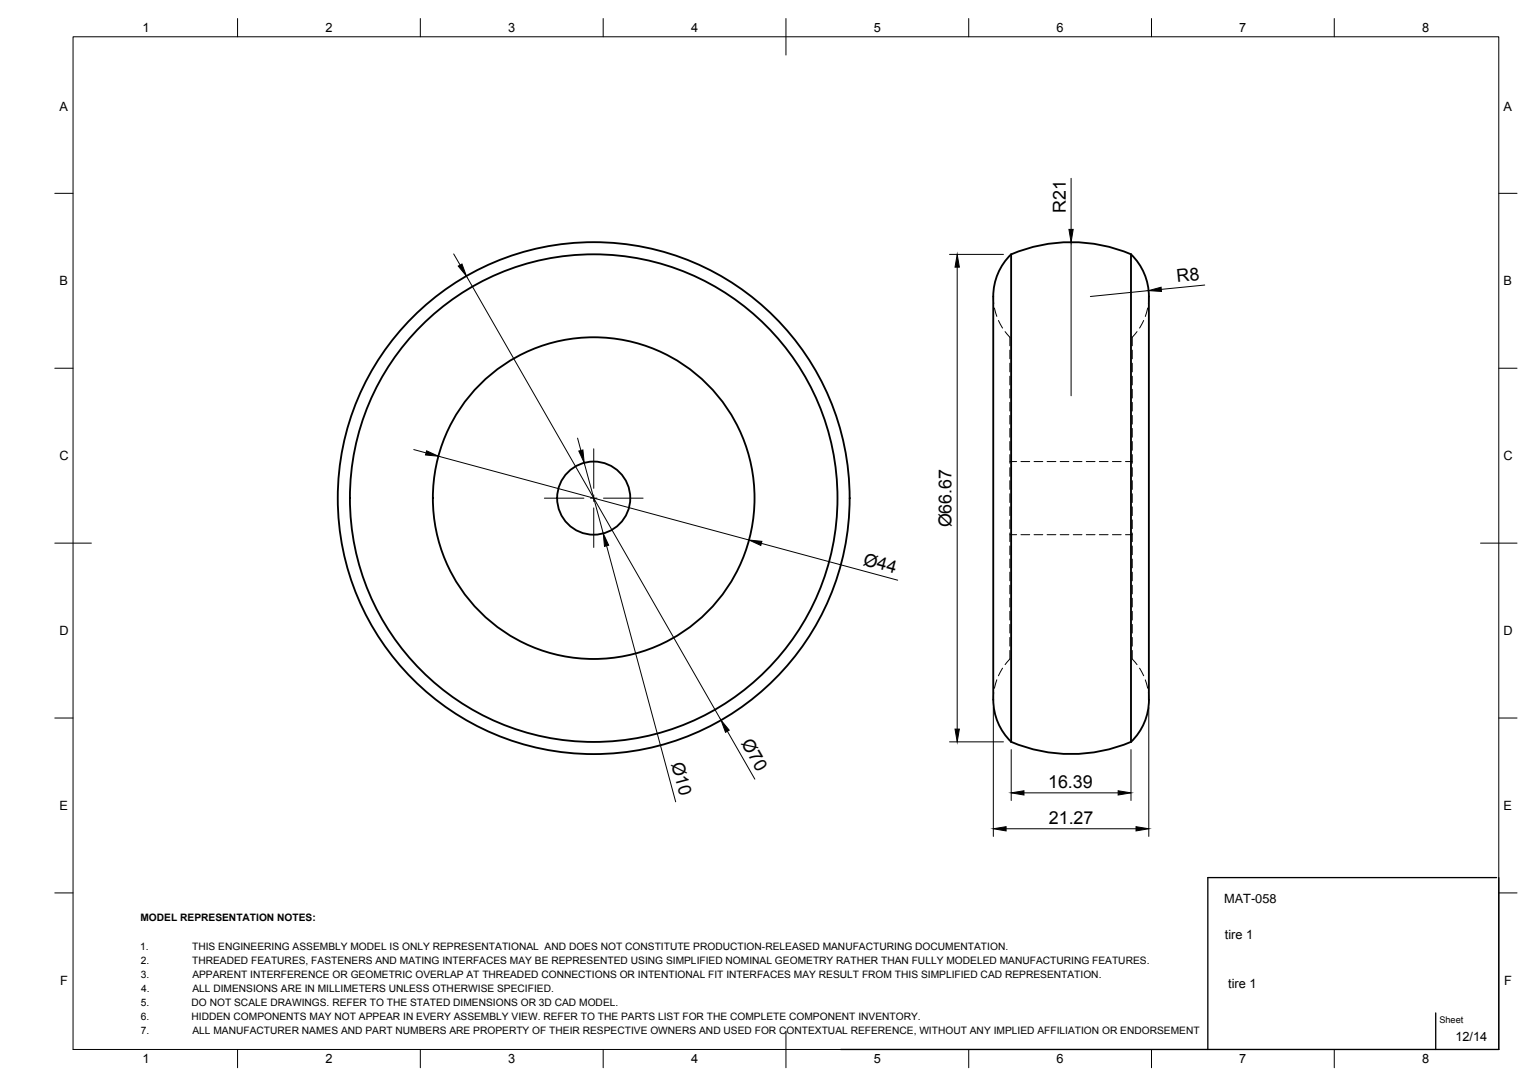
ISO-10303-21;
HEADER;
FILE_DESCRIPTION (('STEP AP214'),
    '1' );
FILE_NAME ('tire 1.step',
    '2026-10-21T17:54:40',
    ( '' ),
    ( '' ),
    'SwSTEP 2.0',
    'SolidWorks 2026',
    '' );
FILE_SCHEMA (( 'AUTOMOTIVE_DESIGN' ));
ENDSEC;

DATA;
#3=ORIENTED_EDGE ( 'NONE', *, *, #134, .T. ) ;
#134=EDGE_CURVE ( 'NONE', #24013, #25229, #8136, .T. ) ;
#450=PRODUCT_DEFINITION_FORMATION_WITH_SPECIFIED_SOURCE ( 'ANY', '', #29832, .NOT_KNOWN. ) ;
#461=DIRECTION ( 'NONE',  ( -1.000000000000000000, -0.000000000000000000, -0.000000000000000000 ) ) ;
#822=DIRECTION ( 'NONE',  ( -1.000000000000000000, -0.000000000000000000, -0.000000000000000000 ) ) ;
#883=ADVANCED_FACE ( 'NONE', ( #35791 ), #3095, .T. ) ;
#885=AXIS2_PLACEMENT_3D ( 'NONE', #24920, #14879, #22568 ) ;
#1237=VERTEX_POINT ( 'NONE', #11074 ) ;
#1353=DIRECTION ( 'NONE',  ( 0.000000000000000000, -1.224646799147352961E-16, 1.000000000000000000 ) ) ;
#1445=FACE_OUTER_BOUND ( 'NONE', #37012, .T. ) ;
#1633=CIRCLE ( 'NONE', #43400, 22.00000000000000000 ) ;
#1686=DIRECTION ( 'NONE',  ( -1.000000000000000000, -0.000000000000000000, -0.000000000000000000 ) ) ;
#2253=ORIENTED_EDGE ( 'NONE', *, *, #43738, .T. ) ;
#3057=DIRECTION ( 'NONE',  ( 0.000000000000000000, 0.000000000000000000, 1.000000000000000000 ) ) ;
#3095=TOROIDAL_SURFACE ( 'NONE', #31808, 27.58190990837850265, 8.000000000000000000 ) ;
#3153=CLOSED_SHELL ( 'NONE', ( #5898, #9220, #18286, #37671, #20586, #18104, #14876, #883, #26048, #41307 ) ) ;
#3617=CARTESIAN_POINT ( 'NONE',  ( -1.642172164747307761, 0.000000000000000000, 27.58190990837850265 ) ) ;
#3941=EDGE_CURVE ( 'NONE', #40207, #1237, #47400, .T. ) ;
#4194=VERTEX_POINT ( 'NONE', #39222 ) ;
#4266=( LENGTH_UNIT ( ) NAMED_UNIT ( * ) SI_UNIT ( .MILLI., .METRE. ) );
#4521=DIRECTION ( 'NONE',  ( 0.000000000000000000, 0.000000000000000000, -1.000000000000000000 ) ) ;
#4589=AXIS2_PLACEMENT_3D ( 'NONE', #21174, #1686, #4521 ) ;
#4597=DIRECTION ( 'NONE',  ( 0.000000000000000000, 0.000000000000000000, 1.000000000000000000 ) ) ;
#4997=VERTEX_POINT ( 'NONE', #45113 ) ;
#5069=DIRECTION ( 'NONE',  ( 0.000000000000000000, 0.000000000000000000, -1.000000000000000000 ) ) ;
#5073=UNCERTAINTY_MEASURE_WITH_UNIT (LENGTH_MEASURE( 1.000000000000000082E-05 ), #4266, 'distance_accuracy_value', 'NONE');
#5186=CARTESIAN_POINT ( 'NONE',  ( 3.627208138665139803, 3.377809768366639828E-15, -27.58190990837850265 ) ) ;
#5215=DIRECTION ( 'NONE',  ( -0.000000000000000000, 0.000000000000000000, 1.000000000000000000 ) ) ;
#5308=AXIS2_PLACEMENT_3D ( 'NONE', #16570, #47819, #12711 ) ;
#5438=DIRECTION ( 'NONE',  ( 0.000000000000000000, 0.000000000000000000, -1.000000000000000000 ) ) ;
#5528=DIRECTION ( 'NONE',  ( 0.000000000000000000, -1.224646799147352961E-16, 1.000000000000000000 ) ) ;
#5532=MANIFOLD_SOLID_BREP ( 'Cut-Extrude1', #3153 ) ;
#5590=VERTEX_POINT ( 'NONE', #17317 ) ;
#5840=CARTESIAN_POINT ( 'NONE',  ( -7.372990760266265653, 0.000000000000000000, 0.000000000000000000 ) ) ;
#5898=ADVANCED_FACE ( 'NONE', ( #44142 ), #37251, .F. ) ;
#5914=ORIENTED_EDGE ( 'NONE', *, *, #13078, .F. ) ;
#6211=DIRECTION ( 'NONE',  ( 1.000000000000000000, 0.000000000000000000, 0.000000000000000000 ) ) ;
#6301=ADVANCED_BREP_SHAPE_REPRESENTATION ( '', ( #5532, #45486 ), #38984 ) ;
#6304=DIRECTION ( 'NONE',  ( -1.000000000000000000, -0.000000000000000000, -0.000000000000000000 ) ) ;
#6817=TOROIDAL_SURFACE ( 'NONE', #21572, 27.58190990837850265, 8.000000000000000000 ) ;
#7306=AXIS2_PLACEMENT_3D ( 'NONE', #34640, #28697, #4597 ) ;
#7375=CIRCLE ( 'NONE', #12277, 20.99999999999999289 ) ;
#7527=ORIENTED_EDGE ( 'NONE', *, *, #40856, .T. ) ;
#7765=TOROIDAL_SURFACE ( 'NONE', #29871, 27.58190990837850265, 8.000000000000000000 ) ;
#7813=DIRECTION ( 'NONE',  ( 0.000000000000000000, 0.000000000000000000, 1.000000000000000000 ) ) ;
#8136=CIRCLE ( 'NONE', #47408, 8.000000000000000000 ) ;
#8438=SHAPE_REPRESENTATION ( 'tire 1', ( #45486 ), #38984 ) ;
#8740=CARTESIAN_POINT ( 'NONE',  ( -9.643172164747307207, 6.123233995736766282E-16, 5.000000000000000000 ) ) ;
#9130=DIRECTION ( 'NONE',  ( -0.000000000000000000, 1.000000000000000000, 1.224646799147353207E-16 ) ) ;
#9177=DIRECTION ( 'NONE',  ( 0.000000000000000000, 0.000000000000000000, 1.000000000000000000 ) ) ;
#9220=ADVANCED_FACE ( 'NONE', ( #49094 ), #40899, .T. ) ;
#9304=DIRECTION ( 'NONE',  ( 0.000000000000000000, -1.224646799147353207E-16, 1.000000000000000000 ) ) ;
#9319=FACE_OUTER_BOUND ( 'NONE', #17798, .T. ) ;
#9347=CARTESIAN_POINT ( 'NONE',  ( 9.358026734184097251, 0.000000000000000000, 0.000000000000000000 ) ) ;
#9413=AXIS2_PLACEMENT_3D ( 'NONE', #43306, #23048, #38978 ) ;
#9443=CARTESIAN_POINT ( 'NONE',  ( -7.200076171898729172, 0.000000000000000000, 0.000000000000000000 ) ) ;
#9886=CARTESIAN_POINT ( 'NONE',  ( 3.627208138665139803, 0.000000000000000000, 0.000000000000000000 ) ) ;
#10134=DIRECTION ( 'NONE',  ( 0.000000000000000000, 0.000000000000000000, 1.000000000000000000 ) ) ;
#10168=EDGE_CURVE ( 'NONE', #20400, #29240, #39842, .T. ) ;
#10474=ORIENTED_EDGE ( 'NONE', *, *, #35944, .F. ) ;
#10579=ORIENTED_EDGE ( 'NONE', *, *, #30205, .T. ) ;
#10812=DIRECTION ( 'NONE',  ( 0.000000000000000000, -1.000000000000000000, 0.000000000000000000 ) ) ;
#10904=APPLICATION_CONTEXT ( 'automotive_design' ) ;
#11038=ORIENTED_EDGE ( 'NONE', *, *, #30205, .F. ) ;
#11074=CARTESIAN_POINT ( 'NONE',  ( 9.185112145816566098, 4.082484168683570285E-15, -33.33601305720110020 ) ) ;
#11289=ORIENTED_EDGE ( 'NONE', *, *, #10168, .F. ) ;
#11709=EDGE_CURVE ( 'NONE', #29240, #1237, #26209, .T. ) ;
#11747=DIRECTION ( 'NONE',  ( 0.000000000000000000, 0.000000000000000000, 1.000000000000000000 ) ) ;
#11876=ORIENTED_EDGE ( 'NONE', *, *, #31746, .T. ) ;
#11930=DIRECTION ( 'NONE',  ( 0.000000000000000000, 0.000000000000000000, 1.000000000000000000 ) ) ;
#12005=AXIS2_PLACEMENT_3D ( 'NONE', #25454, #6211, #5438 ) ;
#12277=AXIS2_PLACEMENT_3D ( 'NONE', #28780, #44156, #37267 ) ;
#12476=MECHANICAL_DESIGN_GEOMETRIC_PRESENTATION_REPRESENTATION('',(#29698),#31333);
#12652=PLANE ( 'NONE',  #34799 ) ;
#12682=DIRECTION ( 'NONE',  ( -1.000000000000000000, -0.000000000000000000, -0.000000000000000000 ) ) ;
#12711=DIRECTION ( 'NONE',  ( 0.000000000000000000, 0.000000000000000000, -1.000000000000000000 ) ) ;
#13023=DIRECTION ( 'NONE',  ( -1.000000000000000000, -0.000000000000000000, -0.000000000000000000 ) ) ;
#13078=EDGE_CURVE ( 'NONE', #24013, #18422, #22060, .T. ) ;
#13189=DIRECTION ( 'NONE',  ( 0.000000000000000000, 0.000000000000000000, 1.000000000000000000 ) ) ;
#13288=ORIENTED_EDGE ( 'NONE', *, *, #16440, .F. ) ;
#13319=DIRECTION ( 'NONE',  ( 0.000000000000000000, 0.000000000000000000, 1.000000000000000000 ) ) ;
#13923=EDGE_CURVE ( 'NONE', #29240, #20400, #26964, .T. ) ;
#14061=DIRECTION ( 'NONE',  ( 0.000000000000000000, 0.000000000000000000, 1.000000000000000000 ) ) ;
#14081=CARTESIAN_POINT ( 'NONE',  ( -7.200076171898729172, 0.000000000000000000, 33.33601305720110020 ) ) ;
#14551=ORIENTED_EDGE ( 'NONE', *, *, #29009, .T. ) ;
#14825=ORIENTED_EDGE ( 'NONE', *, *, #35307, .F. ) ;
#14876=ADVANCED_FACE ( 'NONE', ( #19865 ), #22959, .T. ) ;
#14879=DIRECTION ( 'NONE',  ( 1.000000000000000000, -0.000000000000000000, -0.000000000000000000 ) ) ;
#15061=ORIENTED_EDGE ( 'NONE', *, *, #10168, .T. ) ;
#15269=VECTOR ( 'NONE', #40040, 1000.000000000000000 ) ;
#15314=ORIENTED_EDGE ( 'NONE', *, *, #3941, .T. ) ;
#15382=CARTESIAN_POINT ( 'NONE',  ( -1.642172164747307761, 0.000000000000000000, 0.000000000000000000 ) ) ;
#15504=AXIS2_PLACEMENT_3D ( 'NONE', #35980, #822, #43901 ) ;
#15545=AXIS2_PLACEMENT_3D ( 'NONE', #9443, #18582, #37869 ) ;
#15968=ORIENTED_EDGE ( 'NONE', *, *, #42607, .T. ) ;
#16012=DIRECTION ( 'NONE',  ( -1.000000000000000000, -0.000000000000000000, -0.000000000000000000 ) ) ;
#16282=CIRCLE ( 'NONE', #34300, 8.000000000000000000 ) ;
#16316=( NAMED_UNIT ( * ) PLANE_ANGLE_UNIT ( ) SI_UNIT ( $, .RADIAN. ) );
#16418=AXIS2_PLACEMENT_3D ( 'NONE', #43221, #20372, #11930 ) ;
#16440=EDGE_CURVE ( 'NONE', #1237, #18422, #24667, .T. ) ;
#16505=CARTESIAN_POINT ( 'NONE',  ( 0.9925179869589159098, 1.714505518806294835E-15, -14.00000000000000355 ) ) ;
#16570=CARTESIAN_POINT ( 'NONE',  ( -9.643172164747307207, 0.000000000000000000, 0.000000000000000000 ) ) ;
#16649=DIRECTION ( 'NONE',  ( 0.000000000000000000, 0.000000000000000000, -1.000000000000000000 ) ) ;
#17003=DIRECTION ( 'NONE',  ( -0.000000000000000000, 1.000000000000000000, 1.224646799147353207E-16 ) ) ;
#17075=EDGE_LOOP ( 'NONE', ( #34419, #11876, #45667, #18560 ) ) ;
#17317=CARTESIAN_POINT ( 'NONE',  ( 9.358026734184097251, 6.123233995736766282E-16, 5.000000000000000000 ) ) ;
#17668=CARTESIAN_POINT ( 'NONE',  ( -7.372990760266265653, 0.000000000000000000, 0.000000000000000000 ) ) ;
#17798=EDGE_LOOP ( 'NONE', ( #11289, #49239 ) ) ;
#18104=ADVANCED_FACE ( 'NONE', ( #19205 ), #7765, .T. ) ;
#18286=ADVANCED_FACE ( 'NONE', ( #1445 ), #36452, .T. ) ;
#18422=VERTEX_POINT ( 'NONE', #28322 ) ;
#18560=ORIENTED_EDGE ( 'NONE', *, *, #134, .F. ) ;
#18582=DIRECTION ( 'NONE',  ( -1.000000000000000000, -0.000000000000000000, -0.000000000000000000 ) ) ;
#18788=ORIENTED_EDGE ( 'NONE', *, *, #41944, .F. ) ;
#19083=DIRECTION ( 'NONE',  ( 1.000000000000000000, 0.000000000000000000, 0.000000000000000000 ) ) ;
#19205=FACE_OUTER_BOUND ( 'NONE', #24695, .T. ) ;
#19304=UNCERTAINTY_MEASURE_WITH_UNIT (LENGTH_MEASURE( 1.000000000000000082E-05 ), #46750, 'distance_accuracy_value', 'NONE');
#19445=EDGE_LOOP ( 'NONE', ( #18788, #50003 ) ) ;
#19865=FACE_OUTER_BOUND ( 'NONE', #26339, .T. ) ;
#20356=FACE_BOUND ( 'NONE', #25115, .T. ) ;
#20372=DIRECTION ( 'NONE',  ( -1.000000000000000000, -0.000000000000000000, -0.000000000000000000 ) ) ;
#20400=VERTEX_POINT ( 'NONE', #22412 ) ;
#20586=ADVANCED_FACE ( 'NONE', ( #33422, #48995 ), #44667, .F. ) ;
#20605=( NAMED_UNIT ( * ) PLANE_ANGLE_UNIT ( ) SI_UNIT ( $, .RADIAN. ) );
#20750=DIRECTION ( 'NONE',  ( 1.000000000000000000, 0.000000000000000000, 0.000000000000000000 ) ) ;
#20836=DIRECTION ( 'NONE',  ( -0.000000000000000000, 1.000000000000000000, 1.224646799147353207E-16 ) ) ;
#20954=CIRCLE ( 'NONE', #4589, 5.000000000000000000 ) ;
#21174=CARTESIAN_POINT ( 'NONE',  ( -7.372990760266265653, 0.000000000000000000, 0.000000000000000000 ) ) ;
#21278=ORIENTED_EDGE ( 'NONE', *, *, #11709, .T. ) ;
#21298=SHAPE_DEFINITION_REPRESENTATION ( #33939, #8438 ) ;
#21338=ORIENTED_EDGE ( 'NONE', *, *, #40856, .F. ) ;
#21572=AXIS2_PLACEMENT_3D ( 'NONE', #26675, #22561, #3057 ) ;
#22060=CIRCLE ( 'NONE', #7306, 33.33601305720110020 ) ;
#22412=CARTESIAN_POINT ( 'NONE',  ( 9.358026734184097251, 0.000000000000000000, 22.00000000000000000 ) ) ;
#22561=DIRECTION ( 'NONE',  ( -1.000000000000000000, -0.000000000000000000, -0.000000000000000000 ) ) ;
#22568=DIRECTION ( 'NONE',  ( 0.000000000000000000, 0.000000000000000000, -1.000000000000000000 ) ) ;
#22619=ORIENTED_EDGE ( 'NONE', *, *, #29899, .T. ) ;
#22941=CARTESIAN_POINT ( 'NONE',  ( 9.358026734184097251, 0.000000000000000000, 0.000000000000000000 ) ) ;
#22959=TOROIDAL_SURFACE ( 'NONE', #16418, 14.00000000000000355, 20.99999999999999289 ) ;
#23048=DIRECTION ( 'NONE',  ( 0.000000000000000000, -1.000000000000000000, 0.000000000000000000 ) ) ;
#23552=CARTESIAN_POINT ( 'NONE',  ( -7.372990760266265653, 0.000000000000000000, 0.000000000000000000 ) ) ;
#23923=VECTOR ( 'NONE', #25200, 1000.000000000000000 ) ;
#24013=VERTEX_POINT ( 'NONE', #14081 ) ;
#24254=ORIENTED_EDGE ( 'NONE', *, *, #42409, .T. ) ;
#24391=LINE ( 'NONE', #8740, #15269 ) ;
#24530=AXIS2_PLACEMENT_3D ( 'NONE', #32851, #48432, #13319 ) ;
#24667=CIRCLE ( 'NONE', #43514, 20.99999999999999289 ) ;
#24695=EDGE_LOOP ( 'NONE', ( #35086, #34720, #3, #10474 ) ) ;
#24920=CARTESIAN_POINT ( 'NONE',  ( -9.643172164747307207, 0.000000000000000000, 0.000000000000000000 ) ) ;
#24981=AXIS2_PLACEMENT_3D ( 'NONE', #44504, #28624, #10134 ) ;
#25115=EDGE_LOOP ( 'NONE', ( #34240, #37594 ) ) ;
#25200=DIRECTION ( 'NONE',  ( 1.000000000000000000, -0.000000000000000000, -0.000000000000000000 ) ) ;
#25229=VERTEX_POINT ( 'NONE', #35657 ) ;
#25454=CARTESIAN_POINT ( 'NONE',  ( -7.372990760266265653, 0.000000000000000000, 0.000000000000000000 ) ) ;
#25541=CIRCLE ( 'NONE', #28032, 5.000000000000000000 ) ;
#25711=CARTESIAN_POINT ( 'NONE',  ( -9.643172164747307207, 0.000000000000000000, -5.000000000000000000 ) ) ;
#25723=EDGE_LOOP ( 'NONE', ( #40924, #32757, #7527, #11038 ) ) ;
#25796=DIRECTION ( 'NONE',  ( 0.000000000000000000, 0.000000000000000000, 1.000000000000000000 ) ) ;
#26048=ADVANCED_FACE ( 'NONE', ( #20356, #9319 ), #12652, .F. ) ;
#26209=CIRCLE ( 'NONE', #45824, 8.000000000000000000 ) ;
#26339=EDGE_LOOP ( 'NONE', ( #13288, #10579, #43579, #27328 ) ) ;
#26353=EDGE_LOOP ( 'NONE', ( #40654, #27077 ) ) ;
#26673=DIRECTION ( 'NONE',  ( 0.000000000000000000, 0.000000000000000000, 1.000000000000000000 ) ) ;
#26675=CARTESIAN_POINT ( 'NONE',  ( -1.642172164747307761, 0.000000000000000000, 0.000000000000000000 ) ) ;
#26964=CIRCLE ( 'NONE', #15504, 22.00000000000000000 ) ;
#27077=ORIENTED_EDGE ( 'NONE', *, *, #35944, .T. ) ;
#27328=ORIENTED_EDGE ( 'NONE', *, *, #32908, .F. ) ;
#27803=PRODUCT_DEFINITION_CONTEXT ( 'detailed design', #10904, 'design' ) ;
#28032=AXIS2_PLACEMENT_3D ( 'NONE', #22941, #19083, #50348 ) ;
#28089=ORIENTED_EDGE ( 'NONE', *, *, #41944, .T. ) ;
#28322=CARTESIAN_POINT ( 'NONE',  ( -7.200076171898729172, 4.082484168683569496E-15, -33.33601305720110020 ) ) ;
#28382=EDGE_LOOP ( 'NONE', ( #49116, #24254, #2253, #15968 ) ) ;
#28558=SHAPE_REPRESENTATION_RELATIONSHIP ( 'NONE' , 'NONE' ,  #8438, #6301 ) ;
#28608=FACE_OUTER_BOUND ( 'NONE', #28382, .T. ) ;
#28624=DIRECTION ( 'NONE',  ( -1.000000000000000000, -0.000000000000000000, -0.000000000000000000 ) ) ;
#28697=DIRECTION ( 'NONE',  ( -1.000000000000000000, -0.000000000000000000, -0.000000000000000000 ) ) ;
#28757=CARTESIAN_POINT ( 'NONE',  ( 9.358026734184097251, 0.000000000000000000, -5.000000000000000000 ) ) ;
#28780=CARTESIAN_POINT ( 'NONE',  ( 0.9925179869589159098, 0.000000000000000000, 14.00000000000000355 ) ) ;
#29009=EDGE_CURVE ( 'NONE', #4194, #5590, #24391, .T. ) ;
#29240=VERTEX_POINT ( 'NONE', #29736 ) ;
#29271=APPLICATION_CONTEXT ( 'automotive_design' ) ;
#29665=PRODUCT_DEFINITION ( 'UNKNOWN', '', #450, #27803 ) ;
#29698=STYLED_ITEM('',(#50775),#5532);
#29736=CARTESIAN_POINT ( 'NONE',  ( 9.358026734184097251, 3.388353563403873350E-15, -22.00000000000000000 ) ) ;
#29832=PRODUCT ( 'tire 1', 'tire 1', '', ( #39810 ) ) ;
#29871=AXIS2_PLACEMENT_3D ( 'NONE', #15382, #31037, #26673 ) ;
#29899=EDGE_CURVE ( 'NONE', #5590, #46138, #44819, .T. ) ;
#30205=EDGE_CURVE ( 'NONE', #1237, #40207, #40751, .T. ) ;
#31018=ORIENTED_EDGE ( 'NONE', *, *, #43738, .F. ) ;
#31037=DIRECTION ( 'NONE',  ( -1.000000000000000000, -0.000000000000000000, -0.000000000000000000 ) ) ;
#31090=AXIS2_PLACEMENT_3D ( 'NONE', #9886, #6304, #25796 ) ;
#31113=CIRCLE ( 'NONE', #15545, 33.33601305720110020 ) ;
#31333=( GEOMETRIC_REPRESENTATION_CONTEXT ( 3 ) GLOBAL_UNCERTAINTY_ASSIGNED_CONTEXT ( ( #5073 ) ) GLOBAL_UNIT_ASSIGNED_CONTEXT ( ( #4266, #16316, #42994 ) ) REPRESENTATION_CONTEXT ( 'NONE', 'WORKASPACE' ) );
#31377=EDGE_LOOP ( 'NONE', ( #15061, #21278, #35258, #21338 ) ) ;
#31601=CIRCLE ( 'NONE', #38148, 5.000000000000000000 ) ;
#31746=EDGE_CURVE ( 'NONE', #18422, #4997, #16282, .T. ) ;
#31808=AXIS2_PLACEMENT_3D ( 'NONE', #47009, #16012, #39617 ) ;
#31923=CARTESIAN_POINT ( 'NONE',  ( 0.000000000000000000, 0.000000000000000000, 0.000000000000000000 ) ) ;
#32757=ORIENTED_EDGE ( 'NONE', *, *, #13923, .T. ) ;
#32851=CARTESIAN_POINT ( 'NONE',  ( 9.185112145816566098, 0.000000000000000000, 0.000000000000000000 ) ) ;
#32908=EDGE_CURVE ( 'NONE', #18422, #24013, #31113, .T. ) ;
#33422=FACE_BOUND ( 'NONE', #19445, .T. ) ;
#33939=PRODUCT_DEFINITION_SHAPE ( 'NONE', 'NONE',  #29665 ) ;
#34240=ORIENTED_EDGE ( 'NONE', *, *, #42607, .F. ) ;
#34300=AXIS2_PLACEMENT_3D ( 'NONE', #48334, #9130, #5528 ) ;
#34419=ORIENTED_EDGE ( 'NONE', *, *, #13078, .T. ) ;
#34640=CARTESIAN_POINT ( 'NONE',  ( -7.200076171898729172, 0.000000000000000000, 0.000000000000000000 ) ) ;
#34720=ORIENTED_EDGE ( 'NONE', *, *, #32908, .T. ) ;
#34799=AXIS2_PLACEMENT_3D ( 'NONE', #40124, #44694, #5215 ) ;
#35026=DIRECTION ( 'NONE',  ( 1.000000000000000000, 0.000000000000000000, 0.000000000000000000 ) ) ;
#35086=ORIENTED_EDGE ( 'NONE', *, *, #31746, .F. ) ;
#35096=VERTEX_POINT ( 'NONE', #46210 ) ;
#35258=ORIENTED_EDGE ( 'NONE', *, *, #3941, .F. ) ;
#35307=EDGE_CURVE ( 'NONE', #40207, #24013, #7375, .T. ) ;
#35657=CARTESIAN_POINT ( 'NONE',  ( -7.372990760266265653, 0.000000000000000000, 22.00000000000000000 ) ) ;
#35791=FACE_OUTER_BOUND ( 'NONE', #25723, .T. ) ;
#35889=EDGE_CURVE ( 'NONE', #25229, #4997, #1633, .T. ) ;
#35944=EDGE_CURVE ( 'NONE', #4997, #25229, #37712, .T. ) ;
#35980=CARTESIAN_POINT ( 'NONE',  ( 9.358026734184097251, 0.000000000000000000, 0.000000000000000000 ) ) ;
#36452=TOROIDAL_SURFACE ( 'NONE', #24981, 14.00000000000000355, 20.99999999999999289 ) ;
#36521=LINE ( 'NONE', #25711, #23923 ) ;
#36918=CARTESIAN_POINT ( 'NONE',  ( 9.185112145816566098, 0.000000000000000000, 0.000000000000000000 ) ) ;
#36927=AXIS2_PLACEMENT_3D ( 'NONE', #23552, #461, #11747 ) ;
#37012=EDGE_LOOP ( 'NONE', ( #15314, #37656, #5914, #14825 ) ) ;
#37201=DIRECTION ( 'NONE',  ( -1.000000000000000000, -0.000000000000000000, -0.000000000000000000 ) ) ;
#37251=CYLINDRICAL_SURFACE ( 'NONE', #885, 5.000000000000000000 ) ;
#37267=DIRECTION ( 'NONE',  ( 0.000000000000000000, 0.000000000000000000, -1.000000000000000000 ) ) ;
#37594=ORIENTED_EDGE ( 'NONE', *, *, #29899, .F. ) ;
#37656=ORIENTED_EDGE ( 'NONE', *, *, #16440, .T. ) ;
#37671=ADVANCED_FACE ( 'NONE', ( #46392 ), #6817, .T. ) ;
#37712=CIRCLE ( 'NONE', #36927, 22.00000000000000000 ) ;
#37869=DIRECTION ( 'NONE',  ( 0.000000000000000000, 0.000000000000000000, 1.000000000000000000 ) ) ;
#38148=AXIS2_PLACEMENT_3D ( 'NONE', #5840, #13023, #5069 ) ;
#38546=DIRECTION ( 'NONE',  ( 0.000000000000000000, 0.000000000000000000, -1.000000000000000000 ) ) ;
#38652=CARTESIAN_POINT ( 'NONE',  ( 9.185112145816566098, 0.000000000000000000, 33.33601305720110020 ) ) ;
#38978=DIRECTION ( 'NONE',  ( 0.000000000000000000, 0.000000000000000000, -1.000000000000000000 ) ) ;
#38984=( GEOMETRIC_REPRESENTATION_CONTEXT ( 3 ) GLOBAL_UNCERTAINTY_ASSIGNED_CONTEXT ( ( #19304 ) ) GLOBAL_UNIT_ASSIGNED_CONTEXT ( ( #46750, #20605, #44929 ) ) REPRESENTATION_CONTEXT ( 'NONE', 'WORKASPACE' ) );
#39222=CARTESIAN_POINT ( 'NONE',  ( -7.372990760266265653, 6.123233995736766282E-16, 5.000000000000000000 ) ) ;
#39617=DIRECTION ( 'NONE',  ( 0.000000000000000000, 0.000000000000000000, 1.000000000000000000 ) ) ;
#39810=PRODUCT_CONTEXT ( 'NONE', #29271, 'mechanical' ) ;
#39842=CIRCLE ( 'NONE', #47136, 22.00000000000000000 ) ;
#40040=DIRECTION ( 'NONE',  ( 1.000000000000000000, -0.000000000000000000, -0.000000000000000000 ) ) ;
#40124=CARTESIAN_POINT ( 'NONE',  ( 9.358026734184097251, 0.000000000000000000, 0.000000000000000000 ) ) ;
#40207=VERTEX_POINT ( 'NONE', #38652 ) ;
#40654=ORIENTED_EDGE ( 'NONE', *, *, #35889, .T. ) ;
#40751=CIRCLE ( 'NONE', #49708, 33.33601305720110020 ) ;
#40856=EDGE_CURVE ( 'NONE', #20400, #40207, #42187, .T. ) ;
#40899=TOROIDAL_SURFACE ( 'NONE', #31090, 27.58190990837850265, 8.000000000000000000 ) ;
#40924=ORIENTED_EDGE ( 'NONE', *, *, #11709, .F. ) ;
#41307=ADVANCED_FACE ( 'NONE', ( #28608 ), #43752, .F. ) ;
#41423=EDGE_LOOP ( 'NONE', ( #28089, #14551, #22619, #31018 ) ) ;
#41944=EDGE_CURVE ( 'NONE', #35096, #4194, #31601, .T. ) ;
#42187=CIRCLE ( 'NONE', #9413, 8.000000000000000000 ) ;
#42409=EDGE_CURVE ( 'NONE', #4194, #35096, #20954, .T. ) ;
#42607=EDGE_CURVE ( 'NONE', #46138, #5590, #25541, .T. ) ;
#42994=( NAMED_UNIT ( * ) SI_UNIT ( $, .STERADIAN. ) SOLID_ANGLE_UNIT ( ) );
#43221=CARTESIAN_POINT ( 'NONE',  ( 0.9925179869589159098, 0.000000000000000000, 0.000000000000000000 ) ) ;
#43306=CARTESIAN_POINT ( 'NONE',  ( 3.627208138665139803, 0.000000000000000000, 27.58190990837850265 ) ) ;
#43400=AXIS2_PLACEMENT_3D ( 'NONE', #17668, #37201, #14061 ) ;
#43514=AXIS2_PLACEMENT_3D ( 'NONE', #16505, #17003, #9304 ) ;
#43579=ORIENTED_EDGE ( 'NONE', *, *, #35307, .T. ) ;
#43738=EDGE_CURVE ( 'NONE', #35096, #46138, #36521, .T. ) ;
#43752=CYLINDRICAL_SURFACE ( 'NONE', #5308, 5.000000000000000000 ) ;
#43901=DIRECTION ( 'NONE',  ( 0.000000000000000000, 0.000000000000000000, 1.000000000000000000 ) ) ;
#44142=FACE_OUTER_BOUND ( 'NONE', #41423, .T. ) ;
#44156=DIRECTION ( 'NONE',  ( 0.000000000000000000, -1.000000000000000000, 0.000000000000000000 ) ) ;
#44504=CARTESIAN_POINT ( 'NONE',  ( 0.9925179869589159098, 0.000000000000000000, 0.000000000000000000 ) ) ;
#44667=PLANE ( 'NONE',  #12005 ) ;
#44694=DIRECTION ( 'NONE',  ( -1.000000000000000000, 0.000000000000000000, -0.000000000000000000 ) ) ;
#44819=CIRCLE ( 'NONE', #47268, 5.000000000000000000 ) ;
#44929=( NAMED_UNIT ( * ) SI_UNIT ( $, .STERADIAN. ) SOLID_ANGLE_UNIT ( ) );
#45113=CARTESIAN_POINT ( 'NONE',  ( -7.372990760266265653, 3.388353563403873350E-15, -22.00000000000000000 ) ) ;
#45486=AXIS2_PLACEMENT_3D ( 'NONE', #31923, #7813, #35026 ) ;
#45667=ORIENTED_EDGE ( 'NONE', *, *, #35889, .F. ) ;
#45824=AXIS2_PLACEMENT_3D ( 'NONE', #5186, #20836, #1353 ) ;
#46138=VERTEX_POINT ( 'NONE', #28757 ) ;
#46210=CARTESIAN_POINT ( 'NONE',  ( -7.372990760266265653, 0.000000000000000000, -5.000000000000000000 ) ) ;
#46392=FACE_OUTER_BOUND ( 'NONE', #17075, .T. ) ;
#46750=( LENGTH_UNIT ( ) NAMED_UNIT ( * ) SI_UNIT ( .MILLI., .METRE. ) );
#47009=CARTESIAN_POINT ( 'NONE',  ( 3.627208138665139803, 0.000000000000000000, 0.000000000000000000 ) ) ;
#47136=AXIS2_PLACEMENT_3D ( 'NONE', #9347, #12682, #13189 ) ;
#47268=AXIS2_PLACEMENT_3D ( 'NONE', #47910, #20750, #16649 ) ;
#47375=DIRECTION ( 'NONE',  ( -1.000000000000000000, -0.000000000000000000, -0.000000000000000000 ) ) ;
#47400=CIRCLE ( 'NONE', #24530, 33.33601305720110020 ) ;
#47408=AXIS2_PLACEMENT_3D ( 'NONE', #3617, #10812, #38546 ) ;
#47819=DIRECTION ( 'NONE',  ( 1.000000000000000000, -0.000000000000000000, -0.000000000000000000 ) ) ;
#47910=CARTESIAN_POINT ( 'NONE',  ( 9.358026734184097251, 0.000000000000000000, 0.000000000000000000 ) ) ;
#48334=CARTESIAN_POINT ( 'NONE',  ( -1.642172164747307761, 3.377809768366639828E-15, -27.58190990837850265 ) ) ;
#48432=DIRECTION ( 'NONE',  ( -1.000000000000000000, -0.000000000000000000, -0.000000000000000000 ) ) ;
#48995=FACE_OUTER_BOUND ( 'NONE', #26353, .T. ) ;
#49094=FACE_OUTER_BOUND ( 'NONE', #31377, .T. ) ;
#49116=ORIENTED_EDGE ( 'NONE', *, *, #29009, .F. ) ;
#49239=ORIENTED_EDGE ( 'NONE', *, *, #13923, .F. ) ;
#49708=AXIS2_PLACEMENT_3D ( 'NONE', #36918, #47375, #9177 ) ;
#50003=ORIENTED_EDGE ( 'NONE', *, *, #42409, .F. ) ;
#50348=DIRECTION ( 'NONE',  ( 0.000000000000000000, 0.000000000000000000, -1.000000000000000000 ) ) ;
#50769=COLOUR_RGB('Black',0.12,0.14,0.17);
#50770=FILL_AREA_STYLE_COLOUR('',#50769);
#50771=FILL_AREA_STYLE('',(#50770));
#50772=SURFACE_STYLE_FILL_AREA(#50771);
#50773=SURFACE_SIDE_STYLE('',(#50772));
#50774=SURFACE_STYLE_USAGE(.BOTH.,#50773);
#50775=PRESENTATION_STYLE_ASSIGNMENT((#50774));
ENDSEC;
END-ISO-10303-21;
